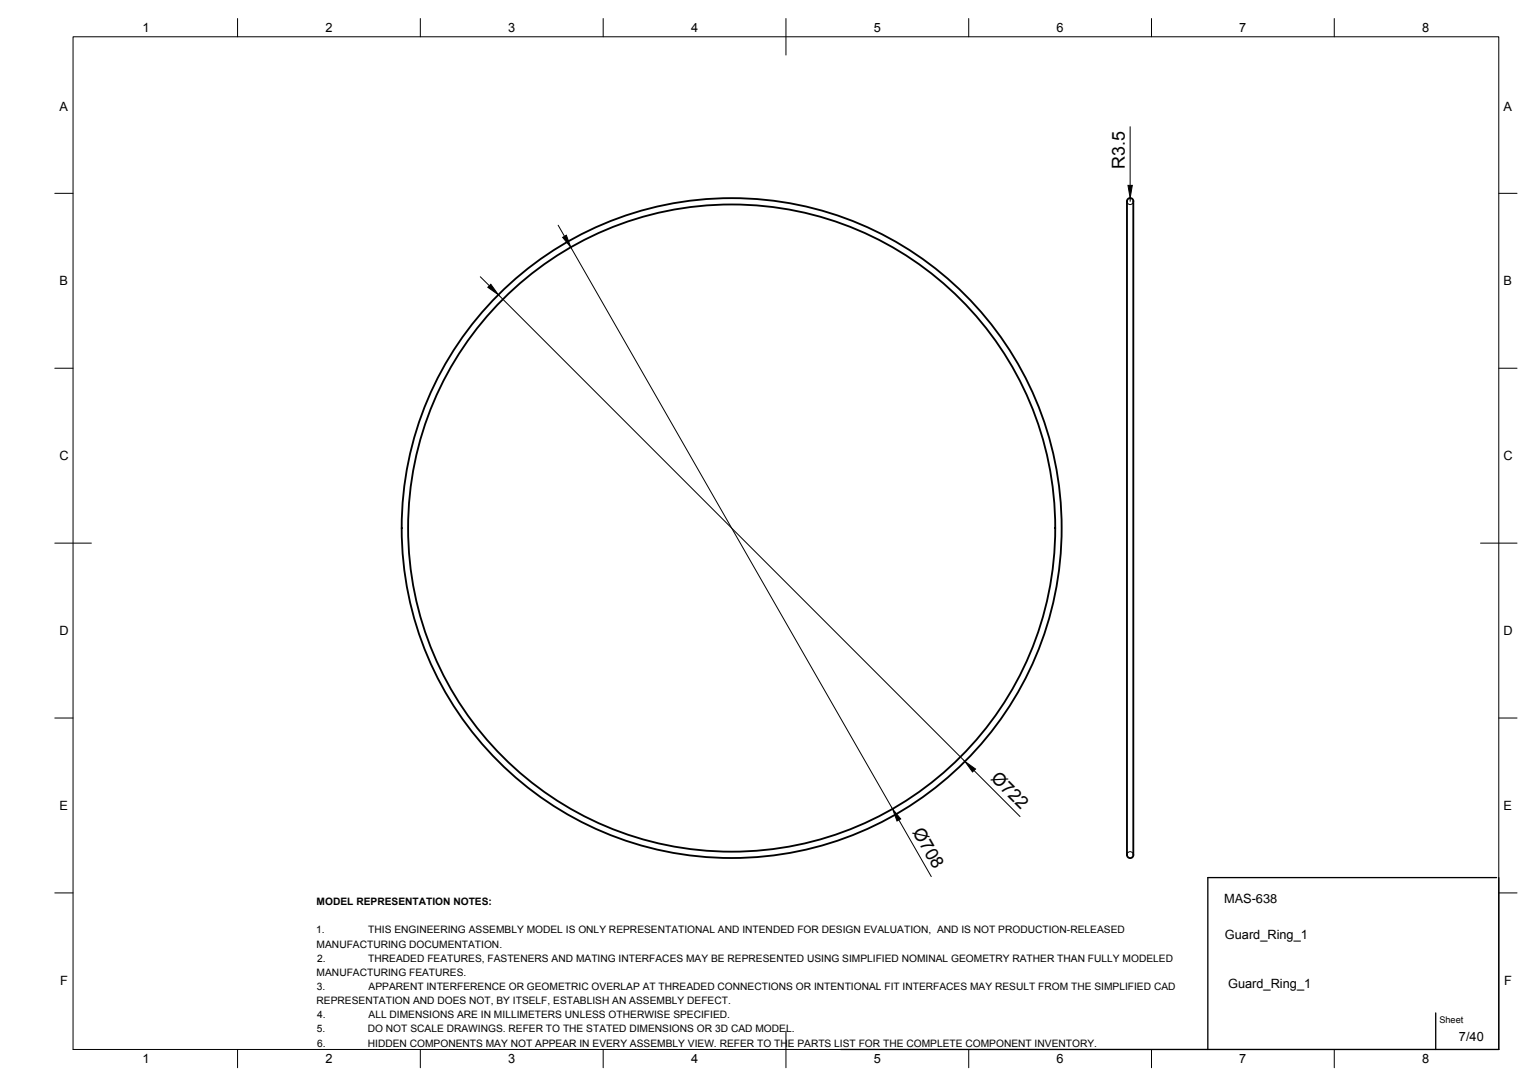
ISO-10303-21;
HEADER;
FILE_DESCRIPTION((''),'2;1');
FILE_NAME('Guard_Ring_1.step','2026-10-09T12:00:21-07:00',(''),(''),'','','');
FILE_SCHEMA (('AUTOMOTIVE_DESIGN { 1 0 10303 214 3 1 1 }'));
ENDSEC;
DATA;
#10=MECHANICAL_DESIGN_GEOMETRIC_PRESENTATION_REPRESENTATION('',(#398),#10334);
#334=SHAPE_REPRESENTATION_RELATIONSHIP('SRR','None',#10450,#366) ;
#366=ADVANCED_BREP_SHAPE_REPRESENTATION('',(#438),#10302) ;
#398=STYLED_ITEM('',(#10631),#438) ;
#438=MANIFOLD_SOLID_BREP('Body1',#3560) ;
#859=FACE_OUTER_BOUND('',#1059,.T.) ;
#1059=EDGE_LOOP('',(#2349,#2350,#2351,#2352)) ;
#1276=CIRCLE('',#3975,0.349999999999999) ;
#1277=CIRCLE('',#3976,35.4) ;
#1513=VERTEX_POINT('',#5653) ;
#1831=EDGE_CURVE('',#1513,#1513,#1276,.T.) ;
#1832=EDGE_CURVE('',#1513,#1513,#1277,.T.) ;
#2349=ORIENTED_EDGE('',*,*,#1831,.F.) ;
#2350=ORIENTED_EDGE('',*,*,#1832,.T.) ;
#2351=ORIENTED_EDGE('',*,*,#1831,.T.) ;
#2352=ORIENTED_EDGE('',*,*,#1832,.F.) ;
#3305=TOROIDAL_SURFACE('',#3974,35.75,0.349999999999999) ;
#3367=ADVANCED_FACE('',(#859),#3305,.T.) ;
#3560=CLOSED_SHELL('',(#3367)) ;
#3973=AXIS2_PLACEMENT_3D('',#5651,#4507,#4508) ;
#3974=AXIS2_PLACEMENT_3D('',#5652,#4509,#4510) ;
#3975=AXIS2_PLACEMENT_3D('',#5654,#4511,#4512) ;
#3976=AXIS2_PLACEMENT_3D('',#5655,#4513,#4514) ;
#4507=DIRECTION('axis',(0.,0.,1.)) ;
#4508=DIRECTION('refdir',(1.,0.,0.)) ;
#4509=DIRECTION('center_axis',(6.42891162084177E-17,1.,1.01883556321148E-16)) ;
#4510=DIRECTION('ref_axis',(-1.,0.,0.)) ;
#4511=DIRECTION('center_axis',(0.,1.01883556321148E-16,-1.)) ;
#4512=DIRECTION('ref_axis',(1.,0.,0.)) ;
#4513=DIRECTION('center_axis',(-6.42891162084177E-17,-1.,-1.01883556321148E-16)) ;
#4514=DIRECTION('ref_axis',(-1.,6.42891162084177E-17,6.55000379205715E-33)) ;
#5651=CARTESIAN_POINT('',(0.,0.,0.)) ;
#5652=CARTESIAN_POINT('Origin',(23.47768801576,60.3830586252741,68.2224337400009)) ;
#5653=CARTESIAN_POINT('',(58.87768801576,60.3830586252741,68.2224337400009)) ;
#5654=CARTESIAN_POINT('Origin',(59.22768801576,60.3830586252741,68.2224337400009)) ;
#5655=CARTESIAN_POINT('Origin',(23.47768801576,60.3830586252741,68.2224337400009)) ;
#10265=UNCERTAINTY_MEASURE_WITH_UNIT(LENGTH_MEASURE(0.001),#10335,
'DISTANCE_ACCURACY_VALUE',
'Maximum model space distance between geometric entities at asserted c
onnectivities') ;
#10297=UNCERTAINTY_MEASURE_WITH_UNIT(LENGTH_MEASURE(0.001),#10335,
'DISTANCE_ACCURACY_VALUE',
'Maximum model space distance between geometric entities at asserted c
onnectivities') ;
#10302=(
GEOMETRIC_REPRESENTATION_CONTEXT(3)
GLOBAL_UNCERTAINTY_ASSIGNED_CONTEXT((#10265))
GLOBAL_UNIT_ASSIGNED_CONTEXT((#10335,#10337,#10338))
REPRESENTATION_CONTEXT('','3D')
) ;
#10334=(
GEOMETRIC_REPRESENTATION_CONTEXT(3)
GLOBAL_UNCERTAINTY_ASSIGNED_CONTEXT((#10297))
GLOBAL_UNIT_ASSIGNED_CONTEXT((#10335,#10337,#10338))
REPRESENTATION_CONTEXT('','3D')
) ;
#10335=(
LENGTH_UNIT()
NAMED_UNIT(*)
SI_UNIT(.CENTI.,.METRE.)
) ;
#10337=(
NAMED_UNIT(*)
PLANE_ANGLE_UNIT()
SI_UNIT($,.RADIAN.)
) ;
#10338=(
NAMED_UNIT(*)
SI_UNIT($,.STERADIAN.)
SOLID_ANGLE_UNIT()
) ;
#10343=SHAPE_DEFINITION_REPRESENTATION(#10379,#10450) ;
#10379=PRODUCT_DEFINITION_SHAPE('',$,#10487) ;
#10450=SHAPE_REPRESENTATION('',(#3973),#10302) ;
#10482=PRODUCT_DEFINITION_CONTEXT('part definition',#10592,'design') ;
#10487=PRODUCT_DEFINITION('Guard_Ring_1','Guard_Ring_1',#10523,#10482) ;
#10523=PRODUCT_DEFINITION_FORMATION('',$,#10598) ;
#10592=APPLICATION_CONTEXT(
'Core Data for Automotive Mechanical Design Process') ;
#10593=PRODUCT_CONTEXT('part definition',#10592,'mechanical') ;
#10598=PRODUCT('Guard_Ring_1','Guard_Ring_1',$,(#10593)) ;
#10631=PRESENTATION_STYLE_ASSIGNMENT((#10635)) ;
#10635=SURFACE_STYLE_USAGE(.BOTH.,#10639) ;
#10639=SURFACE_SIDE_STYLE('',(#10643)) ;
#10643=SURFACE_STYLE_FILL_AREA(#10647) ;
#10647=FILL_AREA_STYLE('Opaque(25,25,25)',(#10651)) ;
#10651=FILL_AREA_STYLE_COLOUR('Opaque(25,25,25)',#10655) ;
#10655=COLOUR_RGB('Opaque(25,25,25)', 0.09019608, 0.27058824, 0.51372549) ;
ENDSEC;
END-ISO-10303-21;
